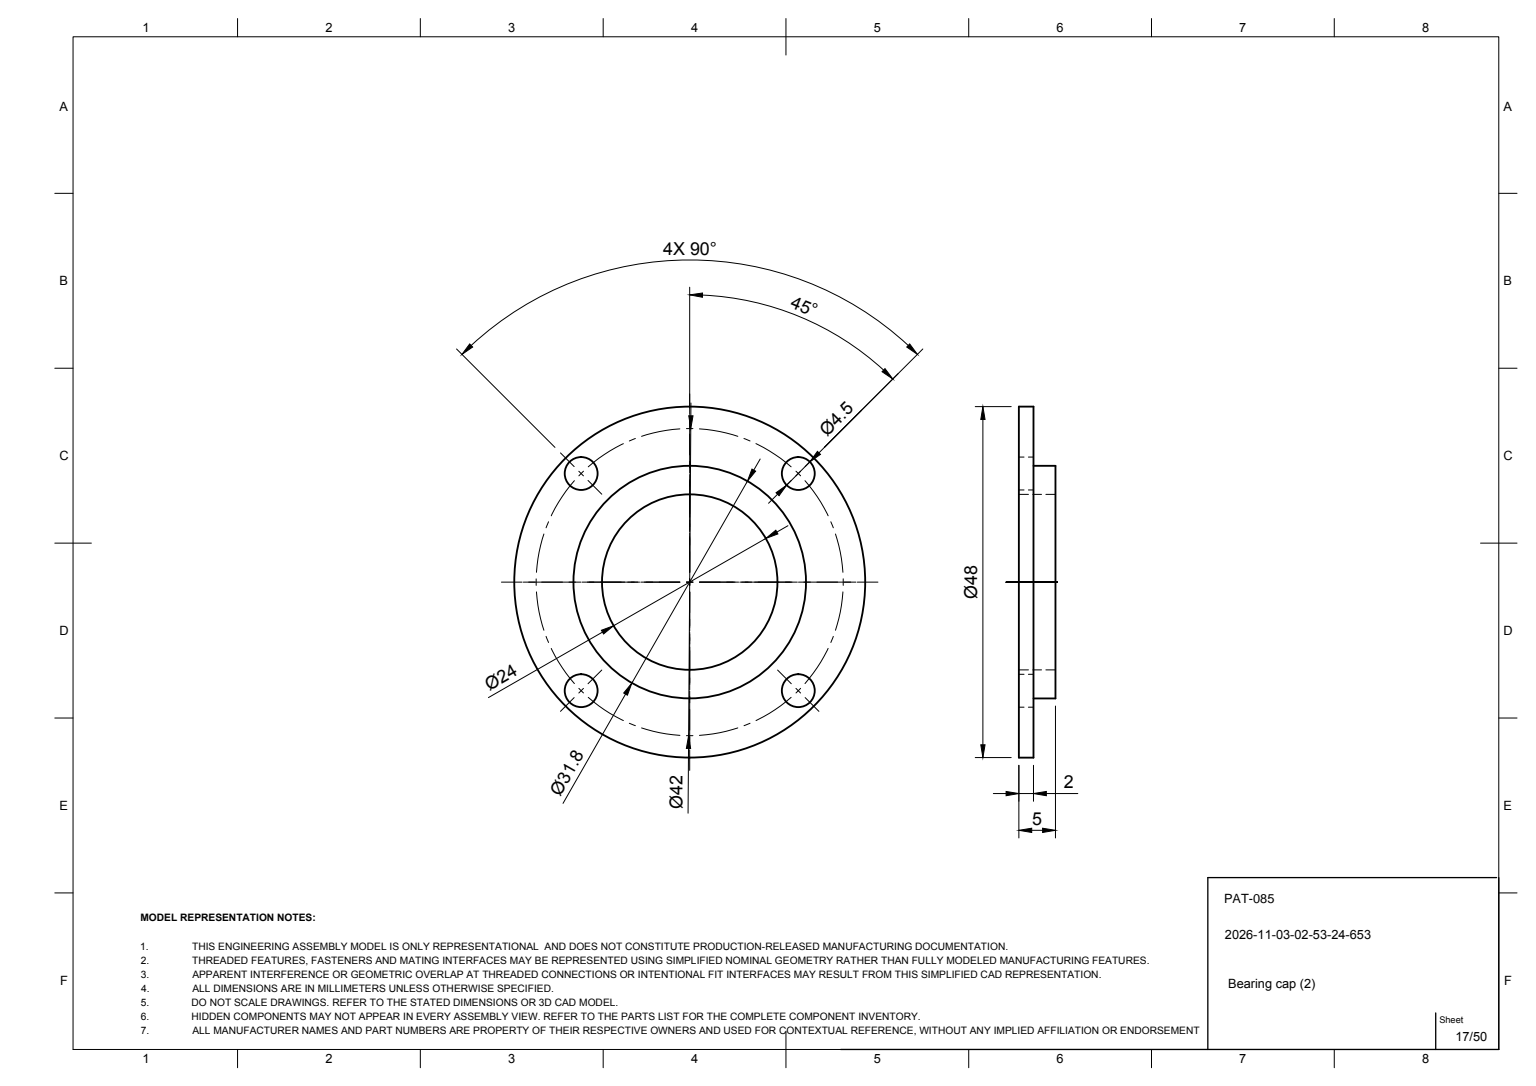
ISO-10303-21;
HEADER;
/* Generated by software containing ST-Developer
 * from STEP Tools, Inc. (www.steptools.com) 
 */

FILE_DESCRIPTION(
/* description */ ('Rack and pinion manual slide'),
/* implementation_level */ '2;1');

FILE_NAME(
/* name */ 'Bearing cap (2).step',
/* time_stamp */ '2026-10-28T03:22:49-07:00',
/* author */ (''),
/* organization */ (''),
/* preprocessor_version */ 'ST-DEVELOPER v20.2',
/* originating_system */ 'Autodesk Translation Framework v15.17.0.0',
/* authorisation */ '');

FILE_SCHEMA (('AUTOMOTIVE_DESIGN { 1 0 10303 214 3 1 1 }'));
ENDSEC;

DATA;
#10=MECHANICAL_DESIGN_GEOMETRIC_PRESENTATION_REPRESENTATION('',(#744),#34851);
#652=SHAPE_REPRESENTATION_RELATIONSHIP('SRR','None',#35087,#698);
#698=ADVANCED_BREP_SHAPE_REPRESENTATION('',(#797),#34812);
#744=STYLED_ITEM('',(#35411),#797);
#797=MANIFOLD_SOLID_BREP('Body1',#13764);
#935=FACE_BOUND('',#2516,.T.);
#936=FACE_BOUND('',#2520,.T.);
#937=FACE_BOUND('',#2521,.T.);
#938=FACE_BOUND('',#2522,.T.);
#939=FACE_BOUND('',#2523,.T.);
#940=FACE_BOUND('',#2524,.T.);
#941=FACE_BOUND('',#2526,.T.);
#942=FACE_BOUND('',#2527,.T.);
#943=FACE_BOUND('',#2528,.T.);
#944=FACE_BOUND('',#2529,.T.);
#945=FACE_BOUND('',#2530,.T.);
#1122=PLANE('',#14593);
#1123=PLANE('',#14600);
#1124=PLANE('',#14601);
#1669=FACE_OUTER_BOUND('',#2510,.T.);
#1670=FACE_OUTER_BOUND('',#2511,.T.);
#1671=FACE_OUTER_BOUND('',#2512,.T.);
#1672=FACE_OUTER_BOUND('',#2513,.T.);
#1673=FACE_OUTER_BOUND('',#2514,.T.);
#1674=FACE_OUTER_BOUND('',#2515,.T.);
#1675=FACE_OUTER_BOUND('',#2517,.T.);
#1676=FACE_OUTER_BOUND('',#2518,.T.);
#1677=FACE_OUTER_BOUND('',#2519,.T.);
#1678=FACE_OUTER_BOUND('',#2525,.T.);
#2510=EDGE_LOOP('',(#9858,#9859,#9860,#9861));
#2511=EDGE_LOOP('',(#9862,#9863,#9864,#9865));
#2512=EDGE_LOOP('',(#9866,#9867,#9868,#9869));
#2513=EDGE_LOOP('',(#9870,#9871,#9872,#9873));
#2514=EDGE_LOOP('',(#9874,#9875,#9876,#9877));
#2515=EDGE_LOOP('',(#9878));
#2516=EDGE_LOOP('',(#9879));
#2517=EDGE_LOOP('',(#9880,#9881,#9882,#9883));
#2518=EDGE_LOOP('',(#9884,#9885,#9886,#9887));
#2519=EDGE_LOOP('',(#9888));
#2520=EDGE_LOOP('',(#9889));
#2521=EDGE_LOOP('',(#9890));
#2522=EDGE_LOOP('',(#9891));
#2523=EDGE_LOOP('',(#9892));
#2524=EDGE_LOOP('',(#9893));
#2525=EDGE_LOOP('',(#9894));
#2526=EDGE_LOOP('',(#9895));
#2527=EDGE_LOOP('',(#9896));
#2528=EDGE_LOOP('',(#9897));
#2529=EDGE_LOOP('',(#9898));
#2530=EDGE_LOOP('',(#9899));
#3424=LINE('',#20130,#4715);
#3425=LINE('',#20136,#4716);
#3426=LINE('',#20142,#4717);
#3427=LINE('',#20148,#4718);
#3428=LINE('',#20154,#4719);
#3429=LINE('',#20161,#4720);
#3430=LINE('',#20167,#4721);
#4715=VECTOR('',#16326,0.225);
#4716=VECTOR('',#16333,0.225);
#4717=VECTOR('',#16340,0.225);
#4718=VECTOR('',#16347,0.225);
#4719=VECTOR('',#16354,1.59);
#4720=VECTOR('',#16363,1.2);
#4721=VECTOR('',#16370,2.4);
#5918=CIRCLE('',#14579,0.225);
#5919=CIRCLE('',#14580,0.225);
#5920=CIRCLE('',#14582,0.225);
#5921=CIRCLE('',#14583,0.225);
#5922=CIRCLE('',#14585,0.225);
#5923=CIRCLE('',#14586,0.225);
#5924=CIRCLE('',#14588,0.225);
#5925=CIRCLE('',#14589,0.225);
#5926=CIRCLE('',#14591,1.59);
#5927=CIRCLE('',#14592,1.59);
#5928=CIRCLE('',#14594,1.2);
#5929=CIRCLE('',#14596,1.2);
#5930=CIRCLE('',#14598,2.4);
#5931=CIRCLE('',#14599,2.4);
#6432=VERTEX_POINT('',#20127);
#6433=VERTEX_POINT('',#20129);
#6434=VERTEX_POINT('',#20133);
#6435=VERTEX_POINT('',#20135);
#6436=VERTEX_POINT('',#20139);
#6437=VERTEX_POINT('',#20141);
#6438=VERTEX_POINT('',#20145);
#6439=VERTEX_POINT('',#20147);
#6440=VERTEX_POINT('',#20151);
#6441=VERTEX_POINT('',#20153);
#6442=VERTEX_POINT('',#20157);
#6443=VERTEX_POINT('',#20160);
#6444=VERTEX_POINT('',#20164);
#6445=VERTEX_POINT('',#20166);
#7741=EDGE_CURVE('',#6432,#6432,#5918,.T.);
#7742=EDGE_CURVE('',#6432,#6433,#3424,.T.);
#7743=EDGE_CURVE('',#6433,#6433,#5919,.T.);
#7744=EDGE_CURVE('',#6434,#6434,#5920,.T.);
#7745=EDGE_CURVE('',#6434,#6435,#3425,.T.);
#7746=EDGE_CURVE('',#6435,#6435,#5921,.T.);
#7747=EDGE_CURVE('',#6436,#6436,#5922,.T.);
#7748=EDGE_CURVE('',#6436,#6437,#3426,.T.);
#7749=EDGE_CURVE('',#6437,#6437,#5923,.T.);
#7750=EDGE_CURVE('',#6438,#6438,#5924,.T.);
#7751=EDGE_CURVE('',#6438,#6439,#3427,.T.);
#7752=EDGE_CURVE('',#6439,#6439,#5925,.T.);
#7753=EDGE_CURVE('',#6440,#6440,#5926,.T.);
#7754=EDGE_CURVE('',#6440,#6441,#3428,.T.);
#7755=EDGE_CURVE('',#6441,#6441,#5927,.T.);
#7756=EDGE_CURVE('',#6442,#6442,#5928,.T.);
#7757=EDGE_CURVE('',#6442,#6443,#3429,.T.);
#7758=EDGE_CURVE('',#6443,#6443,#5929,.T.);
#7759=EDGE_CURVE('',#6444,#6444,#5930,.T.);
#7760=EDGE_CURVE('',#6444,#6445,#3430,.T.);
#7761=EDGE_CURVE('',#6445,#6445,#5931,.T.);
#9858=ORIENTED_EDGE('',*,*,#7741,.F.);
#9859=ORIENTED_EDGE('',*,*,#7742,.T.);
#9860=ORIENTED_EDGE('',*,*,#7743,.F.);
#9861=ORIENTED_EDGE('',*,*,#7742,.F.);
#9862=ORIENTED_EDGE('',*,*,#7744,.F.);
#9863=ORIENTED_EDGE('',*,*,#7745,.T.);
#9864=ORIENTED_EDGE('',*,*,#7746,.F.);
#9865=ORIENTED_EDGE('',*,*,#7745,.F.);
#9866=ORIENTED_EDGE('',*,*,#7747,.F.);
#9867=ORIENTED_EDGE('',*,*,#7748,.T.);
#9868=ORIENTED_EDGE('',*,*,#7749,.F.);
#9869=ORIENTED_EDGE('',*,*,#7748,.F.);
#9870=ORIENTED_EDGE('',*,*,#7750,.F.);
#9871=ORIENTED_EDGE('',*,*,#7751,.T.);
#9872=ORIENTED_EDGE('',*,*,#7752,.F.);
#9873=ORIENTED_EDGE('',*,*,#7751,.F.);
#9874=ORIENTED_EDGE('',*,*,#7753,.F.);
#9875=ORIENTED_EDGE('',*,*,#7754,.T.);
#9876=ORIENTED_EDGE('',*,*,#7755,.F.);
#9877=ORIENTED_EDGE('',*,*,#7754,.F.);
#9878=ORIENTED_EDGE('',*,*,#7753,.T.);
#9879=ORIENTED_EDGE('',*,*,#7756,.T.);
#9880=ORIENTED_EDGE('',*,*,#7756,.F.);
#9881=ORIENTED_EDGE('',*,*,#7757,.T.);
#9882=ORIENTED_EDGE('',*,*,#7758,.T.);
#9883=ORIENTED_EDGE('',*,*,#7757,.F.);
#9884=ORIENTED_EDGE('',*,*,#7759,.F.);
#9885=ORIENTED_EDGE('',*,*,#7760,.T.);
#9886=ORIENTED_EDGE('',*,*,#7761,.T.);
#9887=ORIENTED_EDGE('',*,*,#7760,.F.);
#9888=ORIENTED_EDGE('',*,*,#7759,.T.);
#9889=ORIENTED_EDGE('',*,*,#7755,.T.);
#9890=ORIENTED_EDGE('',*,*,#7752,.T.);
#9891=ORIENTED_EDGE('',*,*,#7749,.T.);
#9892=ORIENTED_EDGE('',*,*,#7746,.T.);
#9893=ORIENTED_EDGE('',*,*,#7743,.T.);
#9894=ORIENTED_EDGE('',*,*,#7761,.F.);
#9895=ORIENTED_EDGE('',*,*,#7758,.F.);
#9896=ORIENTED_EDGE('',*,*,#7750,.T.);
#9897=ORIENTED_EDGE('',*,*,#7747,.T.);
#9898=ORIENTED_EDGE('',*,*,#7744,.T.);
#9899=ORIENTED_EDGE('',*,*,#7741,.T.);
#12900=CYLINDRICAL_SURFACE('',#14578,0.225);
#12901=CYLINDRICAL_SURFACE('',#14581,0.225);
#12902=CYLINDRICAL_SURFACE('',#14584,0.225);
#12903=CYLINDRICAL_SURFACE('',#14587,0.225);
#12904=CYLINDRICAL_SURFACE('',#14590,1.59);
#12905=CYLINDRICAL_SURFACE('',#14595,1.2);
#12906=CYLINDRICAL_SURFACE('',#14597,2.4);
#13147=ADVANCED_FACE('',(#1669),#12900,.F.);
#13148=ADVANCED_FACE('',(#1670),#12901,.F.);
#13149=ADVANCED_FACE('',(#1671),#12902,.F.);
#13150=ADVANCED_FACE('',(#1672),#12903,.F.);
#13151=ADVANCED_FACE('',(#1673),#12904,.T.);
#13152=ADVANCED_FACE('',(#1674,#935),#1122,.T.);
#13153=ADVANCED_FACE('',(#1675),#12905,.F.);
#13154=ADVANCED_FACE('',(#1676),#12906,.T.);
#13155=ADVANCED_FACE('',(#1677,#936,#937,#938,#939,#940),#1123,.T.);
#13156=ADVANCED_FACE('',(#1678,#941,#942,#943,#944,#945),#1124,.F.);
#13764=CLOSED_SHELL('',(#13147,#13148,#13149,#13150,#13151,#13152,#13153,
#13154,#13155,#13156));
#14577=AXIS2_PLACEMENT_3D('',#20125,#16320,#16321);
#14578=AXIS2_PLACEMENT_3D('',#20126,#16322,#16323);
#14579=AXIS2_PLACEMENT_3D('',#20128,#16324,#16325);
#14580=AXIS2_PLACEMENT_3D('',#20131,#16327,#16328);
#14581=AXIS2_PLACEMENT_3D('',#20132,#16329,#16330);
#14582=AXIS2_PLACEMENT_3D('',#20134,#16331,#16332);
#14583=AXIS2_PLACEMENT_3D('',#20137,#16334,#16335);
#14584=AXIS2_PLACEMENT_3D('',#20138,#16336,#16337);
#14585=AXIS2_PLACEMENT_3D('',#20140,#16338,#16339);
#14586=AXIS2_PLACEMENT_3D('',#20143,#16341,#16342);
#14587=AXIS2_PLACEMENT_3D('',#20144,#16343,#16344);
#14588=AXIS2_PLACEMENT_3D('',#20146,#16345,#16346);
#14589=AXIS2_PLACEMENT_3D('',#20149,#16348,#16349);
#14590=AXIS2_PLACEMENT_3D('',#20150,#16350,#16351);
#14591=AXIS2_PLACEMENT_3D('',#20152,#16352,#16353);
#14592=AXIS2_PLACEMENT_3D('',#20155,#16355,#16356);
#14593=AXIS2_PLACEMENT_3D('',#20156,#16357,#16358);
#14594=AXIS2_PLACEMENT_3D('',#20158,#16359,#16360);
#14595=AXIS2_PLACEMENT_3D('',#20159,#16361,#16362);
#14596=AXIS2_PLACEMENT_3D('',#20162,#16364,#16365);
#14597=AXIS2_PLACEMENT_3D('',#20163,#16366,#16367);
#14598=AXIS2_PLACEMENT_3D('',#20165,#16368,#16369);
#14599=AXIS2_PLACEMENT_3D('',#20168,#16371,#16372);
#14600=AXIS2_PLACEMENT_3D('',#20169,#16373,#16374);
#14601=AXIS2_PLACEMENT_3D('',#20170,#16375,#16376);
#16320=DIRECTION('axis',(0.,0.,1.));
#16321=DIRECTION('refdir',(1.,0.,0.));
#16322=DIRECTION('center_axis',(0.,1.,0.));
#16323=DIRECTION('ref_axis',(1.,0.,0.));
#16324=DIRECTION('center_axis',(0.,1.,0.));
#16325=DIRECTION('ref_axis',(1.,0.,0.));
#16326=DIRECTION('',(0.,1.,0.));
#16327=DIRECTION('center_axis',(0.,-1.,0.));
#16328=DIRECTION('ref_axis',(1.,0.,0.));
#16329=DIRECTION('center_axis',(0.,1.,0.));
#16330=DIRECTION('ref_axis',(1.,0.,0.));
#16331=DIRECTION('center_axis',(0.,1.,0.));
#16332=DIRECTION('ref_axis',(1.,0.,0.));
#16333=DIRECTION('',(0.,1.,0.));
#16334=DIRECTION('center_axis',(0.,-1.,0.));
#16335=DIRECTION('ref_axis',(1.,0.,0.));
#16336=DIRECTION('center_axis',(0.,1.,0.));
#16337=DIRECTION('ref_axis',(1.,0.,0.));
#16338=DIRECTION('center_axis',(0.,1.,0.));
#16339=DIRECTION('ref_axis',(1.,0.,0.));
#16340=DIRECTION('',(0.,1.,0.));
#16341=DIRECTION('center_axis',(0.,-1.,0.));
#16342=DIRECTION('ref_axis',(1.,0.,0.));
#16343=DIRECTION('center_axis',(0.,1.,0.));
#16344=DIRECTION('ref_axis',(1.,0.,0.));
#16345=DIRECTION('center_axis',(0.,1.,0.));
#16346=DIRECTION('ref_axis',(1.,0.,0.));
#16347=DIRECTION('',(0.,1.,0.));
#16348=DIRECTION('center_axis',(0.,-1.,0.));
#16349=DIRECTION('ref_axis',(1.,0.,0.));
#16350=DIRECTION('center_axis',(0.,1.,0.));
#16351=DIRECTION('ref_axis',(1.,0.,0.));
#16352=DIRECTION('center_axis',(0.,1.,0.));
#16353=DIRECTION('ref_axis',(1.,0.,0.));
#16354=DIRECTION('',(0.,-1.,0.));
#16355=DIRECTION('center_axis',(0.,-1.,0.));
#16356=DIRECTION('ref_axis',(1.,0.,0.));
#16357=DIRECTION('center_axis',(0.,1.,0.));
#16358=DIRECTION('ref_axis',(1.,0.,0.));
#16359=DIRECTION('center_axis',(0.,-1.,0.));
#16360=DIRECTION('ref_axis',(1.,0.,0.));
#16361=DIRECTION('center_axis',(0.,1.,0.));
#16362=DIRECTION('ref_axis',(1.,0.,0.));
#16363=DIRECTION('',(0.,-1.,0.));
#16364=DIRECTION('center_axis',(0.,-1.,0.));
#16365=DIRECTION('ref_axis',(1.,0.,0.));
#16366=DIRECTION('center_axis',(0.,1.,0.));
#16367=DIRECTION('ref_axis',(1.,0.,0.));
#16368=DIRECTION('center_axis',(0.,1.,0.));
#16369=DIRECTION('ref_axis',(1.,0.,0.));
#16370=DIRECTION('',(0.,-1.,0.));
#16371=DIRECTION('center_axis',(0.,1.,0.));
#16372=DIRECTION('ref_axis',(1.,0.,0.));
#16373=DIRECTION('center_axis',(0.,1.,0.));
#16374=DIRECTION('ref_axis',(1.,0.,0.));
#16375=DIRECTION('center_axis',(0.,1.,0.));
#16376=DIRECTION('ref_axis',(1.,0.,0.));
#20125=CARTESIAN_POINT('',(0.,0.,0.));
#20126=CARTESIAN_POINT('Origin',(9.51507575950825,3.1,8.76507575950825));
#20127=CARTESIAN_POINT('',(9.29007575950825,3.2,8.76507575950825));
#20128=CARTESIAN_POINT('Origin',(9.51507575950825,3.2,8.76507575950825));
#20129=CARTESIAN_POINT('',(9.29007575950825,3.4,8.76507575950825));
#20130=CARTESIAN_POINT('',(9.29007575950825,3.1,8.76507575950825));
#20131=CARTESIAN_POINT('Origin',(9.51507575950825,3.4,8.76507575950825));
#20132=CARTESIAN_POINT('Origin',(9.51507575950825,3.1,11.7349242404918));
#20133=CARTESIAN_POINT('',(9.29007575950825,3.2,11.7349242404918));
#20134=CARTESIAN_POINT('Origin',(9.51507575950825,3.2,11.7349242404918));
#20135=CARTESIAN_POINT('',(9.29007575950825,3.4,11.7349242404918));
#20136=CARTESIAN_POINT('',(9.29007575950825,3.1,11.7349242404918));
#20137=CARTESIAN_POINT('Origin',(9.51507575950825,3.4,11.7349242404918));
#20138=CARTESIAN_POINT('Origin',(12.4849242404918,3.1,11.7349242404918));
#20139=CARTESIAN_POINT('',(12.2599242404918,3.2,11.7349242404918));
#20140=CARTESIAN_POINT('Origin',(12.4849242404918,3.2,11.7349242404918));
#20141=CARTESIAN_POINT('',(12.2599242404918,3.4,11.7349242404918));
#20142=CARTESIAN_POINT('',(12.2599242404918,3.1,11.7349242404918));
#20143=CARTESIAN_POINT('Origin',(12.4849242404918,3.4,11.7349242404918));
#20144=CARTESIAN_POINT('Origin',(12.4849242404917,3.1,8.76507575950825));
#20145=CARTESIAN_POINT('',(12.2599242404917,3.2,8.76507575950825));
#20146=CARTESIAN_POINT('Origin',(12.4849242404917,3.2,8.76507575950825));
#20147=CARTESIAN_POINT('',(12.2599242404917,3.4,8.76507575950825));
#20148=CARTESIAN_POINT('',(12.2599242404917,3.1,8.76507575950825));
#20149=CARTESIAN_POINT('Origin',(12.4849242404917,3.4,8.76507575950825));
#20150=CARTESIAN_POINT('Origin',(11.,3.4,10.25));
#20151=CARTESIAN_POINT('',(9.41,3.7,10.25));
#20152=CARTESIAN_POINT('Origin',(11.,3.7,10.25));
#20153=CARTESIAN_POINT('',(9.41,3.4,10.25));
#20154=CARTESIAN_POINT('',(9.41,3.4,10.25));
#20155=CARTESIAN_POINT('Origin',(11.,3.4,10.25));
#20156=CARTESIAN_POINT('Origin',(11.,3.7,10.25));
#20157=CARTESIAN_POINT('',(9.8,3.7,10.25));
#20158=CARTESIAN_POINT('Origin',(11.,3.7,10.25));
#20159=CARTESIAN_POINT('Origin',(11.,3.2,10.25));
#20160=CARTESIAN_POINT('',(9.8,3.2,10.25));
#20161=CARTESIAN_POINT('',(9.8,3.2,10.25));
#20162=CARTESIAN_POINT('Origin',(11.,3.2,10.25));
#20163=CARTESIAN_POINT('Origin',(11.,3.2,10.25));
#20164=CARTESIAN_POINT('',(8.6,3.4,10.25));
#20165=CARTESIAN_POINT('Origin',(11.,3.4,10.25));
#20166=CARTESIAN_POINT('',(8.6,3.2,10.25));
#20167=CARTESIAN_POINT('',(8.6,3.2,10.25));
#20168=CARTESIAN_POINT('Origin',(11.,3.2,10.25));
#20169=CARTESIAN_POINT('Origin',(11.,3.4,10.25));
#20170=CARTESIAN_POINT('Origin',(11.,3.2,10.25));
#34758=UNCERTAINTY_MEASURE_WITH_UNIT(LENGTH_MEASURE(0.001),#34852,
'DISTANCE_ACCURACY_VALUE',
'Maximum model space distance between geometric entities at asserted c
onnectivities');
#34797=UNCERTAINTY_MEASURE_WITH_UNIT(LENGTH_MEASURE(0.001),#34852,
'DISTANCE_ACCURACY_VALUE',
'Maximum model space distance between geometric entities at asserted c
onnectivities');
#34812=(
GEOMETRIC_REPRESENTATION_CONTEXT(3)
GLOBAL_UNCERTAINTY_ASSIGNED_CONTEXT((#34758))
GLOBAL_UNIT_ASSIGNED_CONTEXT((#34852,#34854,#34855))
REPRESENTATION_CONTEXT('','3D')
);
#34851=(
GEOMETRIC_REPRESENTATION_CONTEXT(3)
GLOBAL_UNCERTAINTY_ASSIGNED_CONTEXT((#34797))
GLOBAL_UNIT_ASSIGNED_CONTEXT((#34852,#34854,#34855))
REPRESENTATION_CONTEXT('','3D')
);
#34852=(
LENGTH_UNIT()
NAMED_UNIT(*)
SI_UNIT(.CENTI.,.METRE.)
);
#34854=(
NAMED_UNIT(*)
PLANE_ANGLE_UNIT()
SI_UNIT($,.RADIAN.)
);
#34855=(
NAMED_UNIT(*)
SI_UNIT($,.STERADIAN.)
SOLID_ANGLE_UNIT()
);
#34870=SHAPE_DEFINITION_REPRESENTATION(#34923,#35087);
#34923=PRODUCT_DEFINITION_SHAPE('',$,#35141);
#35087=SHAPE_REPRESENTATION('',(#14577),#34812);
#35126=PRODUCT_DEFINITION_CONTEXT('part definition',#35287,'design');
#35141=PRODUCT_DEFINITION('Bearing cap (2)','Bearing cap (2)',#35194,#35126);
#35194=PRODUCT_DEFINITION_FORMATION('',$,#35303);
#35287=APPLICATION_CONTEXT(
'Core Data for Automotive Mechanical Design Process');
#35288=PRODUCT_CONTEXT('part definition',#35287,'mechanical');
#35303=PRODUCT('Bearing cap (2)','Bearing cap (2)','Bearing cap (2)',(#35288));
#35405=COLOUR_RGB('Grey',0.48,0.52,0.57);
#35406=FILL_AREA_STYLE_COLOUR('',#35405);
#35407=FILL_AREA_STYLE('',(#35406));
#35408=SURFACE_STYLE_FILL_AREA(#35407);
#35409=SURFACE_SIDE_STYLE('',(#35408));
#35410=SURFACE_STYLE_USAGE(.BOTH.,#35409);
#35411=PRESENTATION_STYLE_ASSIGNMENT((#35410));
ENDSEC;
END-ISO-10303-21;
